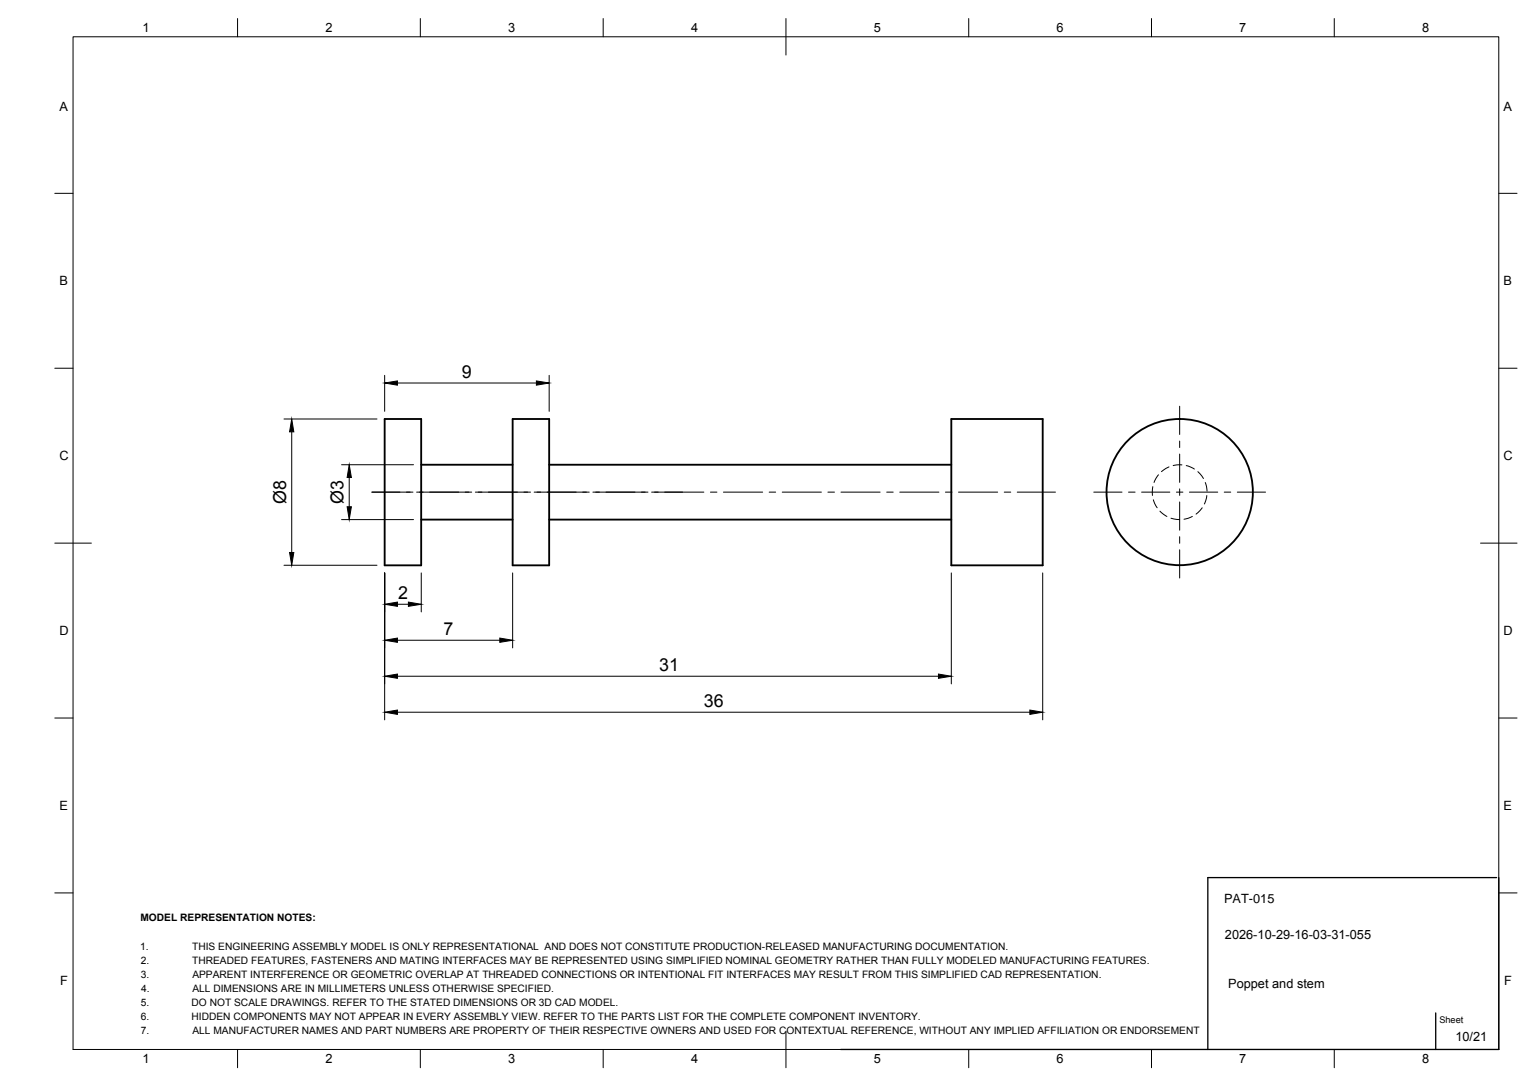
ISO-10303-21;
HEADER;
/* Generated by software containing ST-Developer
 * from STEP Tools, Inc. (www.steptools.com) 
 */

FILE_DESCRIPTION(
/* description */ ('PAT-015'),
/* implementation_level */ '2;1');

FILE_NAME(
/* name */ 'Poppet and stem.step',
/* time_stamp */ '2026-10-29T16:03:43-07:00',
/* author */ (''),
/* organization */ (''),
/* preprocessor_version */ 'ST-DEVELOPER v20.2',
/* originating_system */ 'Autodesk Translation Framework v15.17.0.0',
/* authorisation */ '');

FILE_SCHEMA (('AUTOMOTIVE_DESIGN { 1 0 10303 214 3 1 1 }'));
ENDSEC;

DATA;
#10=MECHANICAL_DESIGN_GEOMETRIC_PRESENTATION_REPRESENTATION('',(#239),#10266);
#191=SHAPE_REPRESENTATION_RELATIONSHIP('SRR','None',#10362,#214);
#214=ADVANCED_BREP_SHAPE_REPRESENTATION('',(#264),#10250);
#239=STYLED_ITEM('',(#10561),#264);
#264=MANIFOLD_SOLID_BREP('Body1',#4698);
#366=FACE_BOUND('',#1066,.T.);
#367=FACE_BOUND('',#1069,.T.);
#368=FACE_BOUND('',#1071,.T.);
#369=FACE_BOUND('',#1078,.T.);
#489=PLANE('',#5232);
#490=PLANE('',#5237);
#491=PLANE('',#5240);
#492=PLANE('',#5247);
#493=PLANE('',#5251);
#494=PLANE('',#5252);
#708=FACE_OUTER_BOUND('',#1065,.T.);
#709=FACE_OUTER_BOUND('',#1067,.T.);
#710=FACE_OUTER_BOUND('',#1068,.T.);
#711=FACE_OUTER_BOUND('',#1070,.T.);
#712=FACE_OUTER_BOUND('',#1072,.T.);
#713=FACE_OUTER_BOUND('',#1073,.T.);
#714=FACE_OUTER_BOUND('',#1074,.T.);
#715=FACE_OUTER_BOUND('',#1075,.T.);
#716=FACE_OUTER_BOUND('',#1076,.T.);
#717=FACE_OUTER_BOUND('',#1077,.T.);
#718=FACE_OUTER_BOUND('',#1079,.T.);
#1065=EDGE_LOOP('',(#3717));
#1066=EDGE_LOOP('',(#3718));
#1067=EDGE_LOOP('',(#3719,#3720,#3721,#3722));
#1068=EDGE_LOOP('',(#3723));
#1069=EDGE_LOOP('',(#3724));
#1070=EDGE_LOOP('',(#3725));
#1071=EDGE_LOOP('',(#3726));
#1072=EDGE_LOOP('',(#3727,#3728,#3729,#3730));
#1073=EDGE_LOOP('',(#3731,#3732,#3733,#3734));
#1074=EDGE_LOOP('',(#3735,#3736,#3737,#3738));
#1075=EDGE_LOOP('',(#3739));
#1076=EDGE_LOOP('',(#3740,#3741,#3742,#3743));
#1077=EDGE_LOOP('',(#3744));
#1078=EDGE_LOOP('',(#3745));
#1079=EDGE_LOOP('',(#3746));
#1461=LINE('',#8701,#1741);
#1462=LINE('',#8713,#1742);
#1463=LINE('',#8716,#1743);
#1464=LINE('',#8719,#1744);
#1465=LINE('',#8725,#1745);
#1741=VECTOR('',#6228,0.4);
#1742=VECTOR('',#6243,0.4);
#1743=VECTOR('',#6246,0.15);
#1744=VECTOR('',#6251,0.15);
#1745=VECTOR('',#6258,0.4);
#1985=CIRCLE('',#5233,0.4);
#1986=CIRCLE('',#5234,0.15);
#1987=CIRCLE('',#5236,0.4);
#1988=CIRCLE('',#5238,0.4);
#1989=CIRCLE('',#5239,0.15);
#1990=CIRCLE('',#5241,0.4);
#1991=CIRCLE('',#5242,0.15);
#1992=CIRCLE('',#5245,0.15);
#1993=CIRCLE('',#5249,0.4);
#1994=CIRCLE('',#5250,0.4);
#2319=VERTEX_POINT('',#8694);
#2320=VERTEX_POINT('',#8696);
#2321=VERTEX_POINT('',#8699);
#2322=VERTEX_POINT('',#8703);
#2323=VERTEX_POINT('',#8705);
#2324=VERTEX_POINT('',#8708);
#2325=VERTEX_POINT('',#8710);
#2326=VERTEX_POINT('',#8715);
#2327=VERTEX_POINT('',#8722);
#2328=VERTEX_POINT('',#8724);
#2814=EDGE_CURVE('',#2319,#2319,#1985,.T.);
#2815=EDGE_CURVE('',#2320,#2320,#1986,.T.);
#2816=EDGE_CURVE('',#2321,#2321,#1987,.T.);
#2817=EDGE_CURVE('',#2321,#2319,#1461,.T.);
#2818=EDGE_CURVE('',#2322,#2322,#1988,.T.);
#2819=EDGE_CURVE('',#2323,#2323,#1989,.T.);
#2820=EDGE_CURVE('',#2324,#2324,#1990,.T.);
#2821=EDGE_CURVE('',#2325,#2325,#1991,.T.);
#2822=EDGE_CURVE('',#2322,#2324,#1462,.T.);
#2823=EDGE_CURVE('',#2325,#2326,#1463,.T.);
#2824=EDGE_CURVE('',#2326,#2326,#1992,.T.);
#2825=EDGE_CURVE('',#2320,#2323,#1464,.T.);
#2826=EDGE_CURVE('',#2327,#2327,#1993,.T.);
#2827=EDGE_CURVE('',#2327,#2328,#1465,.T.);
#2828=EDGE_CURVE('',#2328,#2328,#1994,.T.);
#3717=ORIENTED_EDGE('',*,*,#2814,.F.);
#3718=ORIENTED_EDGE('',*,*,#2815,.F.);
#3719=ORIENTED_EDGE('',*,*,#2816,.F.);
#3720=ORIENTED_EDGE('',*,*,#2817,.T.);
#3721=ORIENTED_EDGE('',*,*,#2814,.T.);
#3722=ORIENTED_EDGE('',*,*,#2817,.F.);
#3723=ORIENTED_EDGE('',*,*,#2818,.T.);
#3724=ORIENTED_EDGE('',*,*,#2819,.F.);
#3725=ORIENTED_EDGE('',*,*,#2820,.F.);
#3726=ORIENTED_EDGE('',*,*,#2821,.F.);
#3727=ORIENTED_EDGE('',*,*,#2818,.F.);
#3728=ORIENTED_EDGE('',*,*,#2822,.T.);
#3729=ORIENTED_EDGE('',*,*,#2820,.T.);
#3730=ORIENTED_EDGE('',*,*,#2822,.F.);
#3731=ORIENTED_EDGE('',*,*,#2821,.T.);
#3732=ORIENTED_EDGE('',*,*,#2823,.T.);
#3733=ORIENTED_EDGE('',*,*,#2824,.F.);
#3734=ORIENTED_EDGE('',*,*,#2823,.F.);
#3735=ORIENTED_EDGE('',*,*,#2815,.T.);
#3736=ORIENTED_EDGE('',*,*,#2825,.T.);
#3737=ORIENTED_EDGE('',*,*,#2819,.T.);
#3738=ORIENTED_EDGE('',*,*,#2825,.F.);
#3739=ORIENTED_EDGE('',*,*,#2816,.T.);
#3740=ORIENTED_EDGE('',*,*,#2826,.F.);
#3741=ORIENTED_EDGE('',*,*,#2827,.T.);
#3742=ORIENTED_EDGE('',*,*,#2828,.T.);
#3743=ORIENTED_EDGE('',*,*,#2827,.F.);
#3744=ORIENTED_EDGE('',*,*,#2826,.T.);
#3745=ORIENTED_EDGE('',*,*,#2824,.T.);
#3746=ORIENTED_EDGE('',*,*,#2828,.F.);
#4356=CYLINDRICAL_SURFACE('',#5235,0.4);
#4357=CYLINDRICAL_SURFACE('',#5243,0.4);
#4358=CYLINDRICAL_SURFACE('',#5244,0.15);
#4359=CYLINDRICAL_SURFACE('',#5246,0.15);
#4360=CYLINDRICAL_SURFACE('',#5248,0.4);
#4543=ADVANCED_FACE('',(#708,#366),#489,.F.);
#4544=ADVANCED_FACE('',(#709),#4356,.T.);
#4545=ADVANCED_FACE('',(#710,#367),#490,.T.);
#4546=ADVANCED_FACE('',(#711,#368),#491,.F.);
#4547=ADVANCED_FACE('',(#712),#4357,.T.);
#4548=ADVANCED_FACE('',(#713),#4358,.T.);
#4549=ADVANCED_FACE('',(#714),#4359,.T.);
#4550=ADVANCED_FACE('',(#715),#492,.T.);
#4551=ADVANCED_FACE('',(#716),#4360,.T.);
#4552=ADVANCED_FACE('',(#717,#369),#493,.T.);
#4553=ADVANCED_FACE('',(#718),#494,.F.);
#4698=CLOSED_SHELL('',(#4543,#4544,#4545,#4546,#4547,#4548,#4549,#4550,
#4551,#4552,#4553));
#5231=AXIS2_PLACEMENT_3D('',#8692,#6216,#6217);
#5232=AXIS2_PLACEMENT_3D('',#8693,#6218,#6219);
#5233=AXIS2_PLACEMENT_3D('',#8695,#6220,#6221);
#5234=AXIS2_PLACEMENT_3D('',#8697,#6222,#6223);
#5235=AXIS2_PLACEMENT_3D('',#8698,#6224,#6225);
#5236=AXIS2_PLACEMENT_3D('',#8700,#6226,#6227);
#5237=AXIS2_PLACEMENT_3D('',#8702,#6229,#6230);
#5238=AXIS2_PLACEMENT_3D('',#8704,#6231,#6232);
#5239=AXIS2_PLACEMENT_3D('',#8706,#6233,#6234);
#5240=AXIS2_PLACEMENT_3D('',#8707,#6235,#6236);
#5241=AXIS2_PLACEMENT_3D('',#8709,#6237,#6238);
#5242=AXIS2_PLACEMENT_3D('',#8711,#6239,#6240);
#5243=AXIS2_PLACEMENT_3D('',#8712,#6241,#6242);
#5244=AXIS2_PLACEMENT_3D('',#8714,#6244,#6245);
#5245=AXIS2_PLACEMENT_3D('',#8717,#6247,#6248);
#5246=AXIS2_PLACEMENT_3D('',#8718,#6249,#6250);
#5247=AXIS2_PLACEMENT_3D('',#8720,#6252,#6253);
#5248=AXIS2_PLACEMENT_3D('',#8721,#6254,#6255);
#5249=AXIS2_PLACEMENT_3D('',#8723,#6256,#6257);
#5250=AXIS2_PLACEMENT_3D('',#8726,#6259,#6260);
#5251=AXIS2_PLACEMENT_3D('',#8727,#6261,#6262);
#5252=AXIS2_PLACEMENT_3D('',#8728,#6263,#6264);
#6216=DIRECTION('axis',(0.,0.,1.));
#6217=DIRECTION('refdir',(1.,0.,0.));
#6218=DIRECTION('center_axis',(0.,0.,1.));
#6219=DIRECTION('ref_axis',(1.,0.,0.));
#6220=DIRECTION('center_axis',(0.,0.,1.));
#6221=DIRECTION('ref_axis',(1.,0.,0.));
#6222=DIRECTION('center_axis',(0.,0.,-1.));
#6223=DIRECTION('ref_axis',(1.,0.,0.));
#6224=DIRECTION('center_axis',(0.,0.,1.));
#6225=DIRECTION('ref_axis',(1.,0.,0.));
#6226=DIRECTION('center_axis',(0.,0.,1.));
#6227=DIRECTION('ref_axis',(1.,0.,0.));
#6228=DIRECTION('',(0.,0.,-1.));
#6229=DIRECTION('center_axis',(0.,0.,1.));
#6230=DIRECTION('ref_axis',(1.,0.,0.));
#6231=DIRECTION('center_axis',(0.,0.,1.));
#6232=DIRECTION('ref_axis',(1.,0.,0.));
#6233=DIRECTION('center_axis',(0.,0.,1.));
#6234=DIRECTION('ref_axis',(1.,0.,0.));
#6235=DIRECTION('center_axis',(0.,0.,1.));
#6236=DIRECTION('ref_axis',(1.,0.,0.));
#6237=DIRECTION('center_axis',(0.,0.,1.));
#6238=DIRECTION('ref_axis',(1.,0.,0.));
#6239=DIRECTION('center_axis',(0.,0.,-1.));
#6240=DIRECTION('ref_axis',(1.,0.,0.));
#6241=DIRECTION('center_axis',(0.,0.,1.));
#6242=DIRECTION('ref_axis',(1.,0.,0.));
#6243=DIRECTION('',(0.,0.,-1.));
#6244=DIRECTION('center_axis',(0.,0.,1.));
#6245=DIRECTION('ref_axis',(1.,0.,0.));
#6246=DIRECTION('',(0.,0.,-1.));
#6247=DIRECTION('center_axis',(0.,0.,-1.));
#6248=DIRECTION('ref_axis',(1.,0.,0.));
#6249=DIRECTION('center_axis',(0.,0.,1.));
#6250=DIRECTION('ref_axis',(1.,0.,0.));
#6251=DIRECTION('',(0.,0.,-1.));
#6252=DIRECTION('center_axis',(0.,0.,1.));
#6253=DIRECTION('ref_axis',(1.,0.,0.));
#6254=DIRECTION('center_axis',(0.,0.,1.));
#6255=DIRECTION('ref_axis',(1.,0.,0.));
#6256=DIRECTION('center_axis',(0.,0.,1.));
#6257=DIRECTION('ref_axis',(1.,0.,0.));
#6258=DIRECTION('',(0.,0.,-1.));
#6259=DIRECTION('center_axis',(0.,0.,1.));
#6260=DIRECTION('ref_axis',(1.,0.,0.));
#6261=DIRECTION('center_axis',(0.,0.,1.));
#6262=DIRECTION('ref_axis',(1.,0.,0.));
#6263=DIRECTION('center_axis',(0.,0.,1.));
#6264=DIRECTION('ref_axis',(1.,0.,0.));
#8692=CARTESIAN_POINT('',(0.,0.,0.));
#8693=CARTESIAN_POINT('Origin',(0.,0.,5.3));
#8694=CARTESIAN_POINT('',(-0.4,-4.89858719658941E-17,5.3));
#8695=CARTESIAN_POINT('Origin',(0.,0.,5.3));
#8696=CARTESIAN_POINT('',(-0.15,1.83697019872103E-17,5.3));
#8697=CARTESIAN_POINT('Origin',(0.,0.,5.3));
#8698=CARTESIAN_POINT('Origin',(0.,0.,5.3));
#8699=CARTESIAN_POINT('',(-0.4,-4.89858719658941E-17,5.5));
#8700=CARTESIAN_POINT('Origin',(0.,0.,5.5));
#8701=CARTESIAN_POINT('',(-0.4,-4.89858719658941E-17,5.3));
#8702=CARTESIAN_POINT('Origin',(0.,0.,4.8));
#8703=CARTESIAN_POINT('',(-0.4,-4.89858719658941E-17,4.8));
#8704=CARTESIAN_POINT('Origin',(0.,0.,4.8));
#8705=CARTESIAN_POINT('',(-0.15,-1.83697019872103E-17,4.8));
#8706=CARTESIAN_POINT('Origin',(0.,0.,4.8));
#8707=CARTESIAN_POINT('Origin',(0.,0.,4.6));
#8708=CARTESIAN_POINT('',(-0.4,-4.89858719658941E-17,4.6));
#8709=CARTESIAN_POINT('Origin',(0.,0.,4.6));
#8710=CARTESIAN_POINT('',(-0.15,1.83697019872103E-17,4.6));
#8711=CARTESIAN_POINT('Origin',(0.,0.,4.6));
#8712=CARTESIAN_POINT('Origin',(0.,0.,4.6));
#8713=CARTESIAN_POINT('',(-0.4,-4.89858719658941E-17,4.6));
#8714=CARTESIAN_POINT('Origin',(0.,0.,2.4));
#8715=CARTESIAN_POINT('',(-0.15,-1.83697019872103E-17,2.4));
#8716=CARTESIAN_POINT('',(-0.15,-1.83697019872103E-17,2.4));
#8717=CARTESIAN_POINT('Origin',(0.,0.,2.4));
#8718=CARTESIAN_POINT('Origin',(0.,0.,2.4));
#8719=CARTESIAN_POINT('',(-0.15,-1.83697019872103E-17,2.4));
#8720=CARTESIAN_POINT('Origin',(0.,0.,5.5));
#8721=CARTESIAN_POINT('Origin',(0.,0.,2.2));
#8722=CARTESIAN_POINT('',(-0.4,-4.89858719658941E-17,2.4));
#8723=CARTESIAN_POINT('Origin',(0.,0.,2.4));
#8724=CARTESIAN_POINT('',(-0.4,-4.89858719658941E-17,1.9));
#8725=CARTESIAN_POINT('',(-0.4,-4.89858719658941E-17,2.2));
#8726=CARTESIAN_POINT('Origin',(0.,0.,1.9));
#8727=CARTESIAN_POINT('Origin',(0.,0.,2.4));
#8728=CARTESIAN_POINT('Origin',(0.,0.,1.9));
#10225=UNCERTAINTY_MEASURE_WITH_UNIT(LENGTH_MEASURE(0.001),#10267,
'DISTANCE_ACCURACY_VALUE',
'Maximum model space distance between geometric entities at asserted c
onnectivities');
#10241=UNCERTAINTY_MEASURE_WITH_UNIT(LENGTH_MEASURE(0.001),#10267,
'DISTANCE_ACCURACY_VALUE',
'Maximum model space distance between geometric entities at asserted c
onnectivities');
#10250=(
GEOMETRIC_REPRESENTATION_CONTEXT(3)
GLOBAL_UNCERTAINTY_ASSIGNED_CONTEXT((#10225))
GLOBAL_UNIT_ASSIGNED_CONTEXT((#10267,#10269,#10270))
REPRESENTATION_CONTEXT('','3D')
);
#10266=(
GEOMETRIC_REPRESENTATION_CONTEXT(3)
GLOBAL_UNCERTAINTY_ASSIGNED_CONTEXT((#10241))
GLOBAL_UNIT_ASSIGNED_CONTEXT((#10267,#10269,#10270))
REPRESENTATION_CONTEXT('','3D')
);
#10267=(
LENGTH_UNIT()
NAMED_UNIT(*)
SI_UNIT(.CENTI.,.METRE.)
);
#10269=(
NAMED_UNIT(*)
PLANE_ANGLE_UNIT()
SI_UNIT($,.RADIAN.)
);
#10270=(
NAMED_UNIT(*)
SI_UNIT($,.STERADIAN.)
SOLID_ANGLE_UNIT()
);
#10279=SHAPE_DEFINITION_REPRESENTATION(#10303,#10362);
#10303=PRODUCT_DEFINITION_SHAPE('',$,#10387);
#10362=SHAPE_REPRESENTATION('',(#5231),#10250);
#10378=PRODUCT_DEFINITION_CONTEXT('part definition',#10452,'design');
#10387=PRODUCT_DEFINITION('Poppet and stem','Poppet and stem',
#10411,#10378);
#10411=PRODUCT_DEFINITION_FORMATION('',$,#10462);
#10452=APPLICATION_CONTEXT(
'Core Data for Automotive Mechanical Design Process');
#10453=PRODUCT_CONTEXT('part definition',#10452,'mechanical');
#10462=PRODUCT('Poppet and stem','Poppet and stem',
'Poppet and stem',(#10453));
#10555=COLOUR_RGB('Off White',0.89,0.88,0.83);
#10556=FILL_AREA_STYLE_COLOUR('',#10555);
#10557=FILL_AREA_STYLE('',(#10556));
#10558=SURFACE_STYLE_FILL_AREA(#10557);
#10559=SURFACE_SIDE_STYLE('',(#10558));
#10560=SURFACE_STYLE_USAGE(.BOTH.,#10559);
#10561=PRESENTATION_STYLE_ASSIGNMENT((#10560));
ENDSEC;
END-ISO-10303-21;
